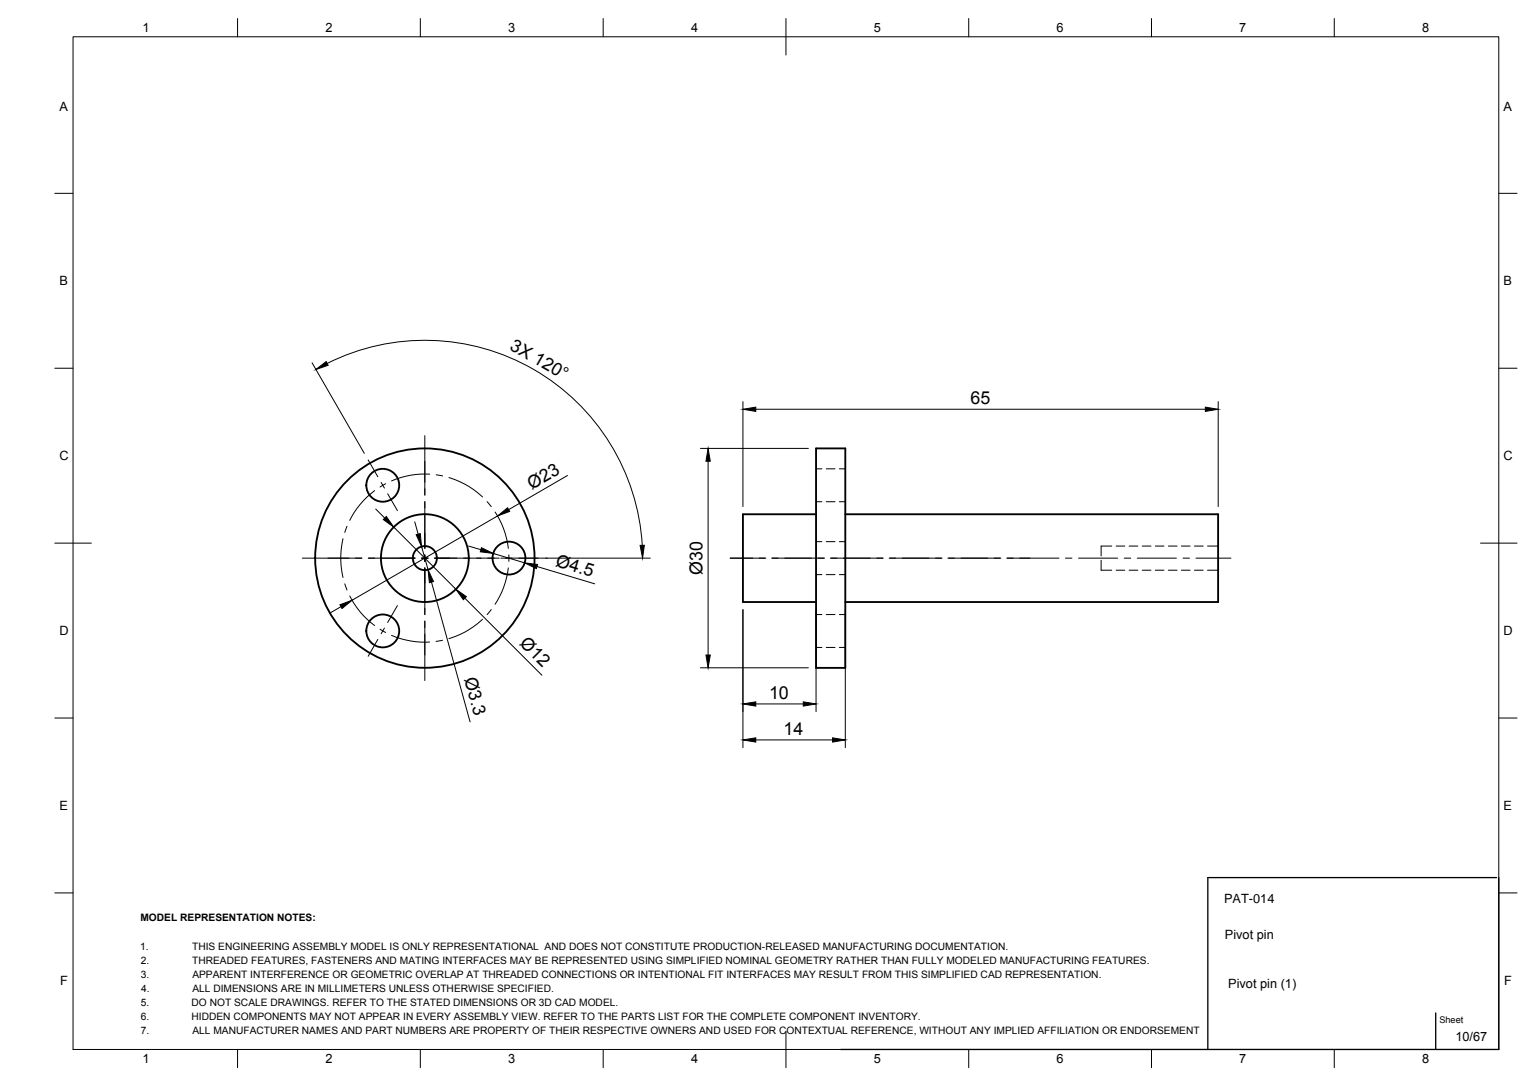
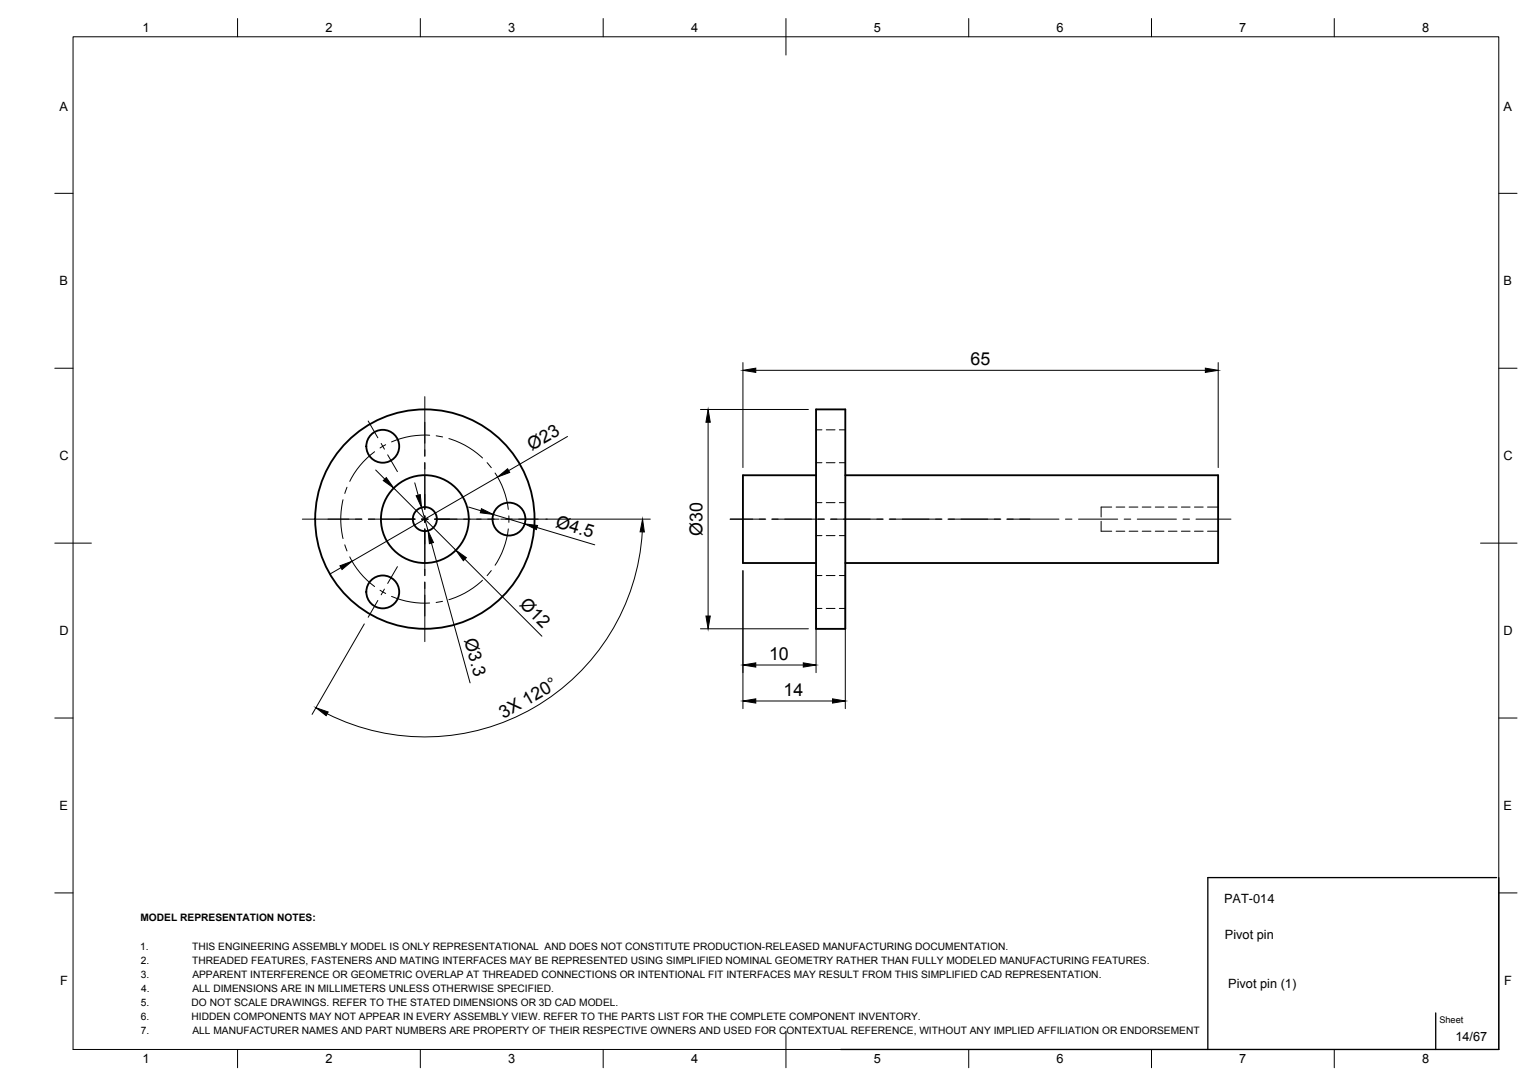
ISO-10303-21;
HEADER;
/* Generated by software containing ST-Developer
 * from STEP Tools, Inc. (www.steptools.com) 
 */

FILE_DESCRIPTION(
/* description */ ('Bin tilter linkage'),
/* implementation_level */ '2;1');

FILE_NAME(
/* name */ 'Pivot pin.step',
/* time_stamp */ '2026-10-28T03:26:24-07:00',
/* author */ (''),
/* organization */ (''),
/* preprocessor_version */ 'ST-DEVELOPER v20.2',
/* originating_system */ 'Autodesk Translation Framework v15.17.0.0',
/* authorisation */ '');

FILE_SCHEMA (('AUTOMOTIVE_DESIGN { 1 0 10303 214 3 1 1 }'));
ENDSEC;

DATA;
#10=MECHANICAL_DESIGN_GEOMETRIC_PRESENTATION_REPRESENTATION('',(#867),#23728);
#655=SHAPE_REPRESENTATION_RELATIONSHIP('SRR','None',#24119,#761);
#761=ADVANCED_BREP_SHAPE_REPRESENTATION('',(#981),#23619);
#867=STYLED_ITEM('',(#24765),#981);
#981=MANIFOLD_SOLID_BREP('Body1',#12397);
#1143=FACE_BOUND('',#2795,.T.);
#1144=FACE_BOUND('',#2796,.T.);
#1145=FACE_BOUND('',#2797,.T.);
#1146=FACE_BOUND('',#2798,.T.);
#1147=FACE_BOUND('',#2800,.T.);
#1148=FACE_BOUND('',#2801,.T.);
#1149=FACE_BOUND('',#2802,.T.);
#1150=FACE_BOUND('',#2803,.T.);
#1151=FACE_BOUND('',#2809,.T.);
#1530=PLANE('',#13809);
#1531=PLANE('',#13819);
#1532=PLANE('',#13822);
#1533=PLANE('',#13830);
#1534=PLANE('',#13831);
#1956=FACE_OUTER_BOUND('',#2789,.T.);
#1957=FACE_OUTER_BOUND('',#2790,.T.);
#1958=FACE_OUTER_BOUND('',#2791,.T.);
#1959=FACE_OUTER_BOUND('',#2792,.T.);
#1960=FACE_OUTER_BOUND('',#2793,.T.);
#1961=FACE_OUTER_BOUND('',#2794,.T.);
#1962=FACE_OUTER_BOUND('',#2799,.T.);
#1963=FACE_OUTER_BOUND('',#2804,.T.);
#1964=FACE_OUTER_BOUND('',#2805,.T.);
#1965=FACE_OUTER_BOUND('',#2806,.T.);
#1966=FACE_OUTER_BOUND('',#2807,.T.);
#1967=FACE_OUTER_BOUND('',#2808,.T.);
#2789=EDGE_LOOP('',(#8709,#8710,#8711,#8712));
#2790=EDGE_LOOP('',(#8713));
#2791=EDGE_LOOP('',(#8714,#8715,#8716,#8717));
#2792=EDGE_LOOP('',(#8718,#8719,#8720,#8721));
#2793=EDGE_LOOP('',(#8722,#8723,#8724,#8725));
#2794=EDGE_LOOP('',(#8726));
#2795=EDGE_LOOP('',(#8727));
#2796=EDGE_LOOP('',(#8728));
#2797=EDGE_LOOP('',(#8729));
#2798=EDGE_LOOP('',(#8730));
#2799=EDGE_LOOP('',(#8731));
#2800=EDGE_LOOP('',(#8732));
#2801=EDGE_LOOP('',(#8733));
#2802=EDGE_LOOP('',(#8734));
#2803=EDGE_LOOP('',(#8735));
#2804=EDGE_LOOP('',(#8736,#8737,#8738,#8739));
#2805=EDGE_LOOP('',(#8740,#8741,#8742,#8743));
#2806=EDGE_LOOP('',(#8744,#8745,#8746,#8747));
#2807=EDGE_LOOP('',(#8748));
#2808=EDGE_LOOP('',(#8749));
#2809=EDGE_LOOP('',(#8750));
#3961=LINE('',#20103,#4636);
#3962=LINE('',#20110,#4637);
#3963=LINE('',#20116,#4638);
#3964=LINE('',#20122,#4639);
#3965=LINE('',#20135,#4640);
#3966=LINE('',#20138,#4641);
#3967=LINE('',#20143,#4642);
#4636=VECTOR('',#15850,0.165);
#4637=VECTOR('',#15859,0.225);
#4638=VECTOR('',#15866,0.225);
#4639=VECTOR('',#15873,0.225);
#4640=VECTOR('',#15890,1.5);
#4641=VECTOR('',#15893,0.6);
#4642=VECTOR('',#15900,0.6);
#5255=CIRCLE('',#13807,0.165);
#5256=CIRCLE('',#13808,0.165);
#5257=CIRCLE('',#13811,0.225);
#5258=CIRCLE('',#13812,0.225);
#5259=CIRCLE('',#13814,0.225);
#5260=CIRCLE('',#13815,0.225);
#5261=CIRCLE('',#13817,0.225);
#5262=CIRCLE('',#13818,0.225);
#5263=CIRCLE('',#13820,1.5);
#5264=CIRCLE('',#13821,0.6);
#5265=CIRCLE('',#13823,1.5);
#5266=CIRCLE('',#13824,0.6);
#5267=CIRCLE('',#13827,0.6);
#5268=CIRCLE('',#13829,0.6);
#6069=VERTEX_POINT('',#20100);
#6070=VERTEX_POINT('',#20102);
#6071=VERTEX_POINT('',#20107);
#6072=VERTEX_POINT('',#20109);
#6073=VERTEX_POINT('',#20113);
#6074=VERTEX_POINT('',#20115);
#6075=VERTEX_POINT('',#20119);
#6076=VERTEX_POINT('',#20121);
#6077=VERTEX_POINT('',#20125);
#6078=VERTEX_POINT('',#20127);
#6079=VERTEX_POINT('',#20130);
#6080=VERTEX_POINT('',#20132);
#6081=VERTEX_POINT('',#20137);
#6082=VERTEX_POINT('',#20141);
#7094=EDGE_CURVE('',#6069,#6069,#5255,.T.);
#7095=EDGE_CURVE('',#6069,#6070,#3961,.T.);
#7096=EDGE_CURVE('',#6070,#6070,#5256,.T.);
#7097=EDGE_CURVE('',#6071,#6071,#5257,.T.);
#7098=EDGE_CURVE('',#6071,#6072,#3962,.T.);
#7099=EDGE_CURVE('',#6072,#6072,#5258,.T.);
#7100=EDGE_CURVE('',#6073,#6073,#5259,.T.);
#7101=EDGE_CURVE('',#6073,#6074,#3963,.T.);
#7102=EDGE_CURVE('',#6074,#6074,#5260,.T.);
#7103=EDGE_CURVE('',#6075,#6075,#5261,.T.);
#7104=EDGE_CURVE('',#6075,#6076,#3964,.T.);
#7105=EDGE_CURVE('',#6076,#6076,#5262,.T.);
#7106=EDGE_CURVE('',#6077,#6077,#5263,.T.);
#7107=EDGE_CURVE('',#6078,#6078,#5264,.T.);
#7108=EDGE_CURVE('',#6079,#6079,#5265,.T.);
#7109=EDGE_CURVE('',#6080,#6080,#5266,.T.);
#7110=EDGE_CURVE('',#6077,#6079,#3965,.T.);
#7111=EDGE_CURVE('',#6080,#6081,#3966,.T.);
#7112=EDGE_CURVE('',#6081,#6081,#5267,.T.);
#7113=EDGE_CURVE('',#6082,#6082,#5268,.T.);
#7114=EDGE_CURVE('',#6082,#6078,#3967,.T.);
#8709=ORIENTED_EDGE('',*,*,#7094,.F.);
#8710=ORIENTED_EDGE('',*,*,#7095,.T.);
#8711=ORIENTED_EDGE('',*,*,#7096,.T.);
#8712=ORIENTED_EDGE('',*,*,#7095,.F.);
#8713=ORIENTED_EDGE('',*,*,#7096,.F.);
#8714=ORIENTED_EDGE('',*,*,#7097,.F.);
#8715=ORIENTED_EDGE('',*,*,#7098,.T.);
#8716=ORIENTED_EDGE('',*,*,#7099,.F.);
#8717=ORIENTED_EDGE('',*,*,#7098,.F.);
#8718=ORIENTED_EDGE('',*,*,#7100,.F.);
#8719=ORIENTED_EDGE('',*,*,#7101,.T.);
#8720=ORIENTED_EDGE('',*,*,#7102,.F.);
#8721=ORIENTED_EDGE('',*,*,#7101,.F.);
#8722=ORIENTED_EDGE('',*,*,#7103,.F.);
#8723=ORIENTED_EDGE('',*,*,#7104,.T.);
#8724=ORIENTED_EDGE('',*,*,#7105,.F.);
#8725=ORIENTED_EDGE('',*,*,#7104,.F.);
#8726=ORIENTED_EDGE('',*,*,#7106,.T.);
#8727=ORIENTED_EDGE('',*,*,#7099,.T.);
#8728=ORIENTED_EDGE('',*,*,#7102,.T.);
#8729=ORIENTED_EDGE('',*,*,#7105,.T.);
#8730=ORIENTED_EDGE('',*,*,#7107,.F.);
#8731=ORIENTED_EDGE('',*,*,#7108,.F.);
#8732=ORIENTED_EDGE('',*,*,#7097,.T.);
#8733=ORIENTED_EDGE('',*,*,#7100,.T.);
#8734=ORIENTED_EDGE('',*,*,#7103,.T.);
#8735=ORIENTED_EDGE('',*,*,#7109,.F.);
#8736=ORIENTED_EDGE('',*,*,#7106,.F.);
#8737=ORIENTED_EDGE('',*,*,#7110,.T.);
#8738=ORIENTED_EDGE('',*,*,#7108,.T.);
#8739=ORIENTED_EDGE('',*,*,#7110,.F.);
#8740=ORIENTED_EDGE('',*,*,#7109,.T.);
#8741=ORIENTED_EDGE('',*,*,#7111,.T.);
#8742=ORIENTED_EDGE('',*,*,#7112,.T.);
#8743=ORIENTED_EDGE('',*,*,#7111,.F.);
#8744=ORIENTED_EDGE('',*,*,#7113,.F.);
#8745=ORIENTED_EDGE('',*,*,#7114,.T.);
#8746=ORIENTED_EDGE('',*,*,#7107,.T.);
#8747=ORIENTED_EDGE('',*,*,#7114,.F.);
#8748=ORIENTED_EDGE('',*,*,#7113,.T.);
#8749=ORIENTED_EDGE('',*,*,#7112,.F.);
#8750=ORIENTED_EDGE('',*,*,#7094,.T.);
#11295=CYLINDRICAL_SURFACE('',#13806,0.165);
#11296=CYLINDRICAL_SURFACE('',#13810,0.225);
#11297=CYLINDRICAL_SURFACE('',#13813,0.225);
#11298=CYLINDRICAL_SURFACE('',#13816,0.225);
#11299=CYLINDRICAL_SURFACE('',#13825,1.5);
#11300=CYLINDRICAL_SURFACE('',#13826,0.6);
#11301=CYLINDRICAL_SURFACE('',#13828,0.6);
#11681=ADVANCED_FACE('',(#1956),#11295,.F.);
#11682=ADVANCED_FACE('',(#1957),#1530,.F.);
#11683=ADVANCED_FACE('',(#1958),#11296,.F.);
#11684=ADVANCED_FACE('',(#1959),#11297,.F.);
#11685=ADVANCED_FACE('',(#1960),#11298,.F.);
#11686=ADVANCED_FACE('',(#1961,#1143,#1144,#1145,#1146),#1531,.T.);
#11687=ADVANCED_FACE('',(#1962,#1147,#1148,#1149,#1150),#1532,.F.);
#11688=ADVANCED_FACE('',(#1963),#11299,.T.);
#11689=ADVANCED_FACE('',(#1964),#11300,.T.);
#11690=ADVANCED_FACE('',(#1965),#11301,.T.);
#11691=ADVANCED_FACE('',(#1966),#1533,.T.);
#11692=ADVANCED_FACE('',(#1967,#1151),#1534,.F.);
#12397=CLOSED_SHELL('',(#11681,#11682,#11683,#11684,#11685,#11686,#11687,
#11688,#11689,#11690,#11691,#11692));
#13805=AXIS2_PLACEMENT_3D('',#20098,#15844,#15845);
#13806=AXIS2_PLACEMENT_3D('',#20099,#15846,#15847);
#13807=AXIS2_PLACEMENT_3D('',#20101,#15848,#15849);
#13808=AXIS2_PLACEMENT_3D('',#20104,#15851,#15852);
#13809=AXIS2_PLACEMENT_3D('',#20105,#15853,#15854);
#13810=AXIS2_PLACEMENT_3D('',#20106,#15855,#15856);
#13811=AXIS2_PLACEMENT_3D('',#20108,#15857,#15858);
#13812=AXIS2_PLACEMENT_3D('',#20111,#15860,#15861);
#13813=AXIS2_PLACEMENT_3D('',#20112,#15862,#15863);
#13814=AXIS2_PLACEMENT_3D('',#20114,#15864,#15865);
#13815=AXIS2_PLACEMENT_3D('',#20117,#15867,#15868);
#13816=AXIS2_PLACEMENT_3D('',#20118,#15869,#15870);
#13817=AXIS2_PLACEMENT_3D('',#20120,#15871,#15872);
#13818=AXIS2_PLACEMENT_3D('',#20123,#15874,#15875);
#13819=AXIS2_PLACEMENT_3D('',#20124,#15876,#15877);
#13820=AXIS2_PLACEMENT_3D('',#20126,#15878,#15879);
#13821=AXIS2_PLACEMENT_3D('',#20128,#15880,#15881);
#13822=AXIS2_PLACEMENT_3D('',#20129,#15882,#15883);
#13823=AXIS2_PLACEMENT_3D('',#20131,#15884,#15885);
#13824=AXIS2_PLACEMENT_3D('',#20133,#15886,#15887);
#13825=AXIS2_PLACEMENT_3D('',#20134,#15888,#15889);
#13826=AXIS2_PLACEMENT_3D('',#20136,#15891,#15892);
#13827=AXIS2_PLACEMENT_3D('',#20139,#15894,#15895);
#13828=AXIS2_PLACEMENT_3D('',#20140,#15896,#15897);
#13829=AXIS2_PLACEMENT_3D('',#20142,#15898,#15899);
#13830=AXIS2_PLACEMENT_3D('',#20144,#15901,#15902);
#13831=AXIS2_PLACEMENT_3D('',#20145,#15903,#15904);
#15844=DIRECTION('axis',(0.,0.,1.));
#15845=DIRECTION('refdir',(1.,0.,0.));
#15846=DIRECTION('center_axis',(0.,1.,0.));
#15847=DIRECTION('ref_axis',(1.,0.,0.));
#15848=DIRECTION('center_axis',(0.,1.,0.));
#15849=DIRECTION('ref_axis',(1.,0.,0.));
#15850=DIRECTION('',(0.,1.,0.));
#15851=DIRECTION('center_axis',(0.,1.,0.));
#15852=DIRECTION('ref_axis',(1.,0.,0.));
#15853=DIRECTION('center_axis',(0.,1.,0.));
#15854=DIRECTION('ref_axis',(1.,0.,0.));
#15855=DIRECTION('center_axis',(0.,1.,0.));
#15856=DIRECTION('ref_axis',(1.,0.,0.));
#15857=DIRECTION('center_axis',(0.,1.,0.));
#15858=DIRECTION('ref_axis',(1.,0.,0.));
#15859=DIRECTION('',(0.,1.,0.));
#15860=DIRECTION('center_axis',(0.,-1.,0.));
#15861=DIRECTION('ref_axis',(1.,0.,0.));
#15862=DIRECTION('center_axis',(0.,1.,0.));
#15863=DIRECTION('ref_axis',(1.,0.,0.));
#15864=DIRECTION('center_axis',(0.,1.,0.));
#15865=DIRECTION('ref_axis',(1.,0.,0.));
#15866=DIRECTION('',(0.,1.,0.));
#15867=DIRECTION('center_axis',(0.,-1.,0.));
#15868=DIRECTION('ref_axis',(1.,0.,0.));
#15869=DIRECTION('center_axis',(0.,1.,0.));
#15870=DIRECTION('ref_axis',(1.,0.,0.));
#15871=DIRECTION('center_axis',(0.,1.,0.));
#15872=DIRECTION('ref_axis',(1.,0.,0.));
#15873=DIRECTION('',(0.,1.,0.));
#15874=DIRECTION('center_axis',(0.,-1.,0.));
#15875=DIRECTION('ref_axis',(1.,0.,0.));
#15876=DIRECTION('center_axis',(0.,1.,0.));
#15877=DIRECTION('ref_axis',(1.,0.,0.));
#15878=DIRECTION('center_axis',(0.,1.,0.));
#15879=DIRECTION('ref_axis',(1.,0.,0.));
#15880=DIRECTION('center_axis',(0.,1.,0.));
#15881=DIRECTION('ref_axis',(1.,0.,0.));
#15882=DIRECTION('center_axis',(0.,1.,0.));
#15883=DIRECTION('ref_axis',(1.,0.,0.));
#15884=DIRECTION('center_axis',(0.,1.,0.));
#15885=DIRECTION('ref_axis',(1.,0.,0.));
#15886=DIRECTION('center_axis',(0.,-1.,0.));
#15887=DIRECTION('ref_axis',(1.,0.,0.));
#15888=DIRECTION('center_axis',(0.,1.,0.));
#15889=DIRECTION('ref_axis',(1.,0.,0.));
#15890=DIRECTION('',(0.,-1.,0.));
#15891=DIRECTION('center_axis',(0.,1.,0.));
#15892=DIRECTION('ref_axis',(1.,0.,0.));
#15893=DIRECTION('',(0.,-1.,0.));
#15894=DIRECTION('center_axis',(0.,1.,0.));
#15895=DIRECTION('ref_axis',(1.,0.,0.));
#15896=DIRECTION('center_axis',(0.,1.,0.));
#15897=DIRECTION('ref_axis',(1.,0.,0.));
#15898=DIRECTION('center_axis',(0.,1.,0.));
#15899=DIRECTION('ref_axis',(1.,0.,0.));
#15900=DIRECTION('',(0.,-1.,0.));
#15901=DIRECTION('center_axis',(0.,1.,0.));
#15902=DIRECTION('ref_axis',(1.,0.,0.));
#15903=DIRECTION('center_axis',(0.,1.,0.));
#15904=DIRECTION('ref_axis',(1.,0.,0.));
#20098=CARTESIAN_POINT('',(0.,0.,0.));
#20099=CARTESIAN_POINT('Origin',(0.,-1.1,15.));
#20100=CARTESIAN_POINT('',(-0.165,-1.,15.));
#20101=CARTESIAN_POINT('Origin',(0.,-1.,15.));
#20102=CARTESIAN_POINT('',(-0.165,0.6,15.));
#20103=CARTESIAN_POINT('',(-0.165,-1.1,15.));
#20104=CARTESIAN_POINT('Origin',(0.,0.6,15.));
#20105=CARTESIAN_POINT('Origin',(0.,0.6,15.));
#20106=CARTESIAN_POINT('Origin',(1.15,4.,15.));
#20107=CARTESIAN_POINT('',(0.925,4.1,15.));
#20108=CARTESIAN_POINT('Origin',(1.15,4.1,15.));
#20109=CARTESIAN_POINT('',(0.925,4.5,15.));
#20110=CARTESIAN_POINT('',(0.925,4.,15.));
#20111=CARTESIAN_POINT('Origin',(1.15,4.5,15.));
#20112=CARTESIAN_POINT('Origin',(-0.575,4.,15.9959292143521));
#20113=CARTESIAN_POINT('',(-0.8,4.1,15.9959292143521));
#20114=CARTESIAN_POINT('Origin',(-0.575,4.1,15.9959292143521));
#20115=CARTESIAN_POINT('',(-0.8,4.5,15.9959292143521));
#20116=CARTESIAN_POINT('',(-0.8,4.,15.9959292143521));
#20117=CARTESIAN_POINT('Origin',(-0.575,4.5,15.9959292143521));
#20118=CARTESIAN_POINT('Origin',(-0.575000000000001,4.,14.0040707856479));
#20119=CARTESIAN_POINT('',(-0.8,4.1,14.0040707856479));
#20120=CARTESIAN_POINT('Origin',(-0.575000000000001,4.1,14.0040707856479));
#20121=CARTESIAN_POINT('',(-0.8,4.5,14.0040707856479));
#20122=CARTESIAN_POINT('',(-0.8,4.,14.0040707856479));
#20123=CARTESIAN_POINT('Origin',(-0.575000000000001,4.5,14.0040707856479));
#20124=CARTESIAN_POINT('Origin',(0.,4.5,15.));
#20125=CARTESIAN_POINT('',(-1.5,4.5,15.));
#20126=CARTESIAN_POINT('Origin',(0.,4.5,15.));
#20127=CARTESIAN_POINT('',(-0.6,4.5,15.));
#20128=CARTESIAN_POINT('Origin',(0.,4.5,15.));
#20129=CARTESIAN_POINT('Origin',(0.,4.1,15.));
#20130=CARTESIAN_POINT('',(-1.5,4.1,15.));
#20131=CARTESIAN_POINT('Origin',(0.,4.1,15.));
#20132=CARTESIAN_POINT('',(-0.6,4.1,15.));
#20133=CARTESIAN_POINT('Origin',(0.,4.1,15.));
#20134=CARTESIAN_POINT('Origin',(0.,4.1,15.));
#20135=CARTESIAN_POINT('',(-1.5,4.1,15.));
#20136=CARTESIAN_POINT('Origin',(0.,-1.,15.));
#20137=CARTESIAN_POINT('',(-0.6,-1.,15.));
#20138=CARTESIAN_POINT('',(-0.6,-1.,15.));
#20139=CARTESIAN_POINT('Origin',(0.,-1.,15.));
#20140=CARTESIAN_POINT('Origin',(0.,-1.,15.));
#20141=CARTESIAN_POINT('',(-0.6,5.5,15.));
#20142=CARTESIAN_POINT('Origin',(0.,5.5,15.));
#20143=CARTESIAN_POINT('',(-0.6,-1.,15.));
#20144=CARTESIAN_POINT('Origin',(0.,5.5,15.));
#20145=CARTESIAN_POINT('Origin',(0.,-1.,15.));
#23502=UNCERTAINTY_MEASURE_WITH_UNIT(LENGTH_MEASURE(0.001),#23729,
'DISTANCE_ACCURACY_VALUE',
'Maximum model space distance between geometric entities at asserted c
onnectivities');
#23611=UNCERTAINTY_MEASURE_WITH_UNIT(LENGTH_MEASURE(0.001),#23729,
'DISTANCE_ACCURACY_VALUE',
'Maximum model space distance between geometric entities at asserted c
onnectivities');
#23619=(
GEOMETRIC_REPRESENTATION_CONTEXT(3)
GLOBAL_UNCERTAINTY_ASSIGNED_CONTEXT((#23502))
GLOBAL_UNIT_ASSIGNED_CONTEXT((#23729,#23731,#23732))
REPRESENTATION_CONTEXT('','3D')
);
#23728=(
GEOMETRIC_REPRESENTATION_CONTEXT(3)
GLOBAL_UNCERTAINTY_ASSIGNED_CONTEXT((#23611))
GLOBAL_UNIT_ASSIGNED_CONTEXT((#23729,#23731,#23732))
REPRESENTATION_CONTEXT('','3D')
);
#23729=(
LENGTH_UNIT()
NAMED_UNIT(*)
SI_UNIT(.CENTI.,.METRE.)
);
#23731=(
NAMED_UNIT(*)
PLANE_ANGLE_UNIT()
SI_UNIT($,.RADIAN.)
);
#23732=(
NAMED_UNIT(*)
SI_UNIT($,.STERADIAN.)
SOLID_ANGLE_UNIT()
);
#23740=SHAPE_DEFINITION_REPRESENTATION(#23856,#24119);
#23856=PRODUCT_DEFINITION_SHAPE('',$,#24236);
#24119=SHAPE_REPRESENTATION('',(#13805),#23619);
#24228=PRODUCT_DEFINITION_CONTEXT('part definition',#24578,'design');
#24236=PRODUCT_DEFINITION('Pivot pin','Pivot pin',#24352,#24228);
#24352=PRODUCT_DEFINITION_FORMATION('',$,#24587);
#24578=APPLICATION_CONTEXT(
'Core Data for Automotive Mechanical Design Process');
#24579=PRODUCT_CONTEXT('part definition',#24578,'mechanical');
#24587=PRODUCT('Pivot pin','Pivot pin','Pivot pin',(#24579));
#24759=COLOUR_RGB('Grey',0.48,0.52,0.57);
#24760=FILL_AREA_STYLE_COLOUR('',#24759);
#24761=FILL_AREA_STYLE('',(#24760));
#24762=SURFACE_STYLE_FILL_AREA(#24761);
#24763=SURFACE_SIDE_STYLE('',(#24762));
#24764=SURFACE_STYLE_USAGE(.BOTH.,#24763);
#24765=PRESENTATION_STYLE_ASSIGNMENT((#24764));
ENDSEC;
END-ISO-10303-21;
